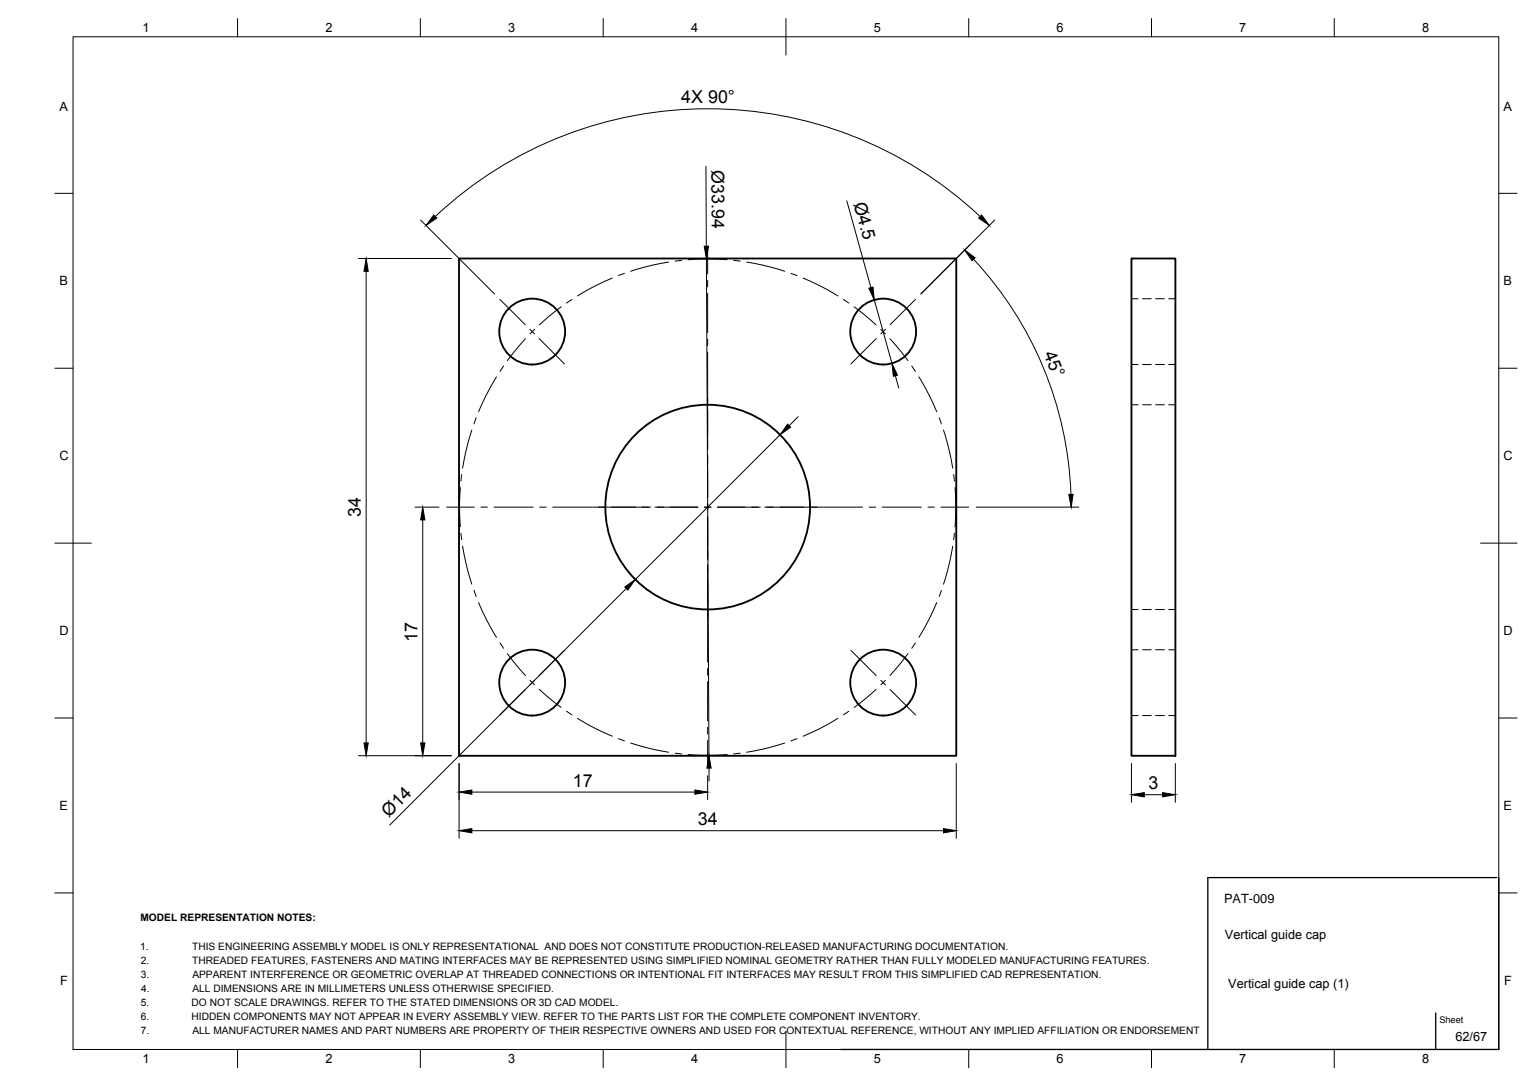
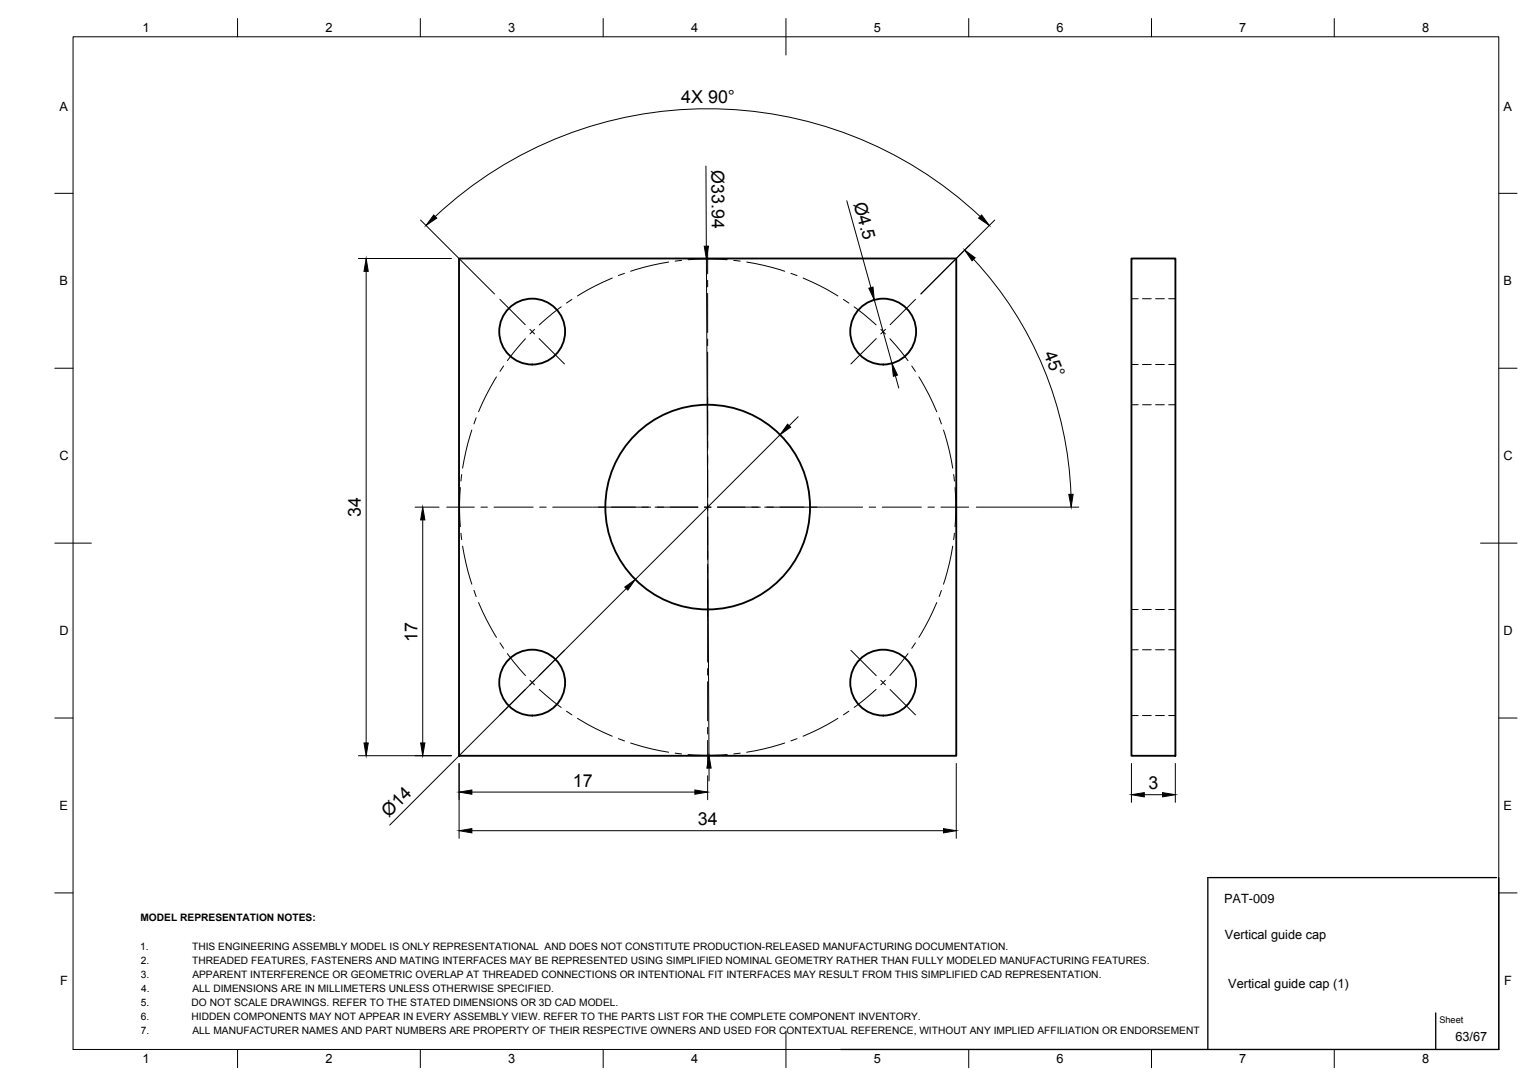
ISO-10303-21;
HEADER;
/* Generated by software containing ST-Developer
 * from STEP Tools, Inc. (www.steptools.com) 
 */

FILE_DESCRIPTION(
/* description */ ('Bell-crank linkage with push rods'),
/* implementation_level */ '2;1');

FILE_NAME(
/* name */ 'Vertical guide cap (1).step',
/* time_stamp */ '2026-10-28T03:25:15-07:00',
/* author */ (''),
/* organization */ (''),
/* preprocessor_version */ 'ST-DEVELOPER v20.2',
/* originating_system */ 'Autodesk Translation Framework v15.17.0.0',
/* authorisation */ '');

FILE_SCHEMA (('AUTOMOTIVE_DESIGN { 1 0 10303 214 3 1 1 }'));
ENDSEC;

DATA;
#10=MECHANICAL_DESIGN_GEOMETRIC_PRESENTATION_REPRESENTATION('',(#658),#16678);
#542=SHAPE_REPRESENTATION_RELATIONSHIP('SRR','None',#16964,#596);
#596=ADVANCED_BREP_SHAPE_REPRESENTATION('',(#718),#16669);
#658=STYLED_ITEM('',(#17277),#718);
#718=MANIFOLD_SOLID_BREP('Body1',#8850);
#935=FACE_BOUND('',#2434,.T.);
#936=FACE_BOUND('',#2435,.T.);
#937=FACE_BOUND('',#2436,.T.);
#938=FACE_BOUND('',#2437,.T.);
#939=FACE_BOUND('',#2438,.T.);
#940=FACE_BOUND('',#2441,.T.);
#941=FACE_BOUND('',#2442,.T.);
#942=FACE_BOUND('',#2443,.T.);
#943=FACE_BOUND('',#2444,.T.);
#944=FACE_BOUND('',#2445,.T.);
#1202=PLANE('',#10415);
#1203=PLANE('',#10416);
#1204=PLANE('',#10417);
#1205=PLANE('',#10418);
#1206=PLANE('',#10419);
#1207=PLANE('',#10420);
#1696=FACE_OUTER_BOUND('',#2428,.T.);
#1697=FACE_OUTER_BOUND('',#2429,.T.);
#1698=FACE_OUTER_BOUND('',#2430,.T.);
#1699=FACE_OUTER_BOUND('',#2431,.T.);
#1700=FACE_OUTER_BOUND('',#2432,.T.);
#1701=FACE_OUTER_BOUND('',#2433,.T.);
#1702=FACE_OUTER_BOUND('',#2439,.T.);
#1703=FACE_OUTER_BOUND('',#2440,.T.);
#1704=FACE_OUTER_BOUND('',#2446,.T.);
#1705=FACE_OUTER_BOUND('',#2447,.T.);
#1706=FACE_OUTER_BOUND('',#2448,.T.);
#2428=EDGE_LOOP('',(#7797,#7798,#7799,#7800));
#2429=EDGE_LOOP('',(#7801,#7802,#7803,#7804));
#2430=EDGE_LOOP('',(#7805,#7806,#7807,#7808));
#2431=EDGE_LOOP('',(#7809,#7810,#7811,#7812));
#2432=EDGE_LOOP('',(#7813,#7814,#7815,#7816));
#2433=EDGE_LOOP('',(#7817,#7818,#7819,#7820));
#2434=EDGE_LOOP('',(#7821));
#2435=EDGE_LOOP('',(#7822));
#2436=EDGE_LOOP('',(#7823));
#2437=EDGE_LOOP('',(#7824));
#2438=EDGE_LOOP('',(#7825));
#2439=EDGE_LOOP('',(#7826,#7827,#7828,#7829));
#2440=EDGE_LOOP('',(#7830,#7831,#7832,#7833));
#2441=EDGE_LOOP('',(#7834));
#2442=EDGE_LOOP('',(#7835));
#2443=EDGE_LOOP('',(#7836));
#2444=EDGE_LOOP('',(#7837));
#2445=EDGE_LOOP('',(#7838));
#2446=EDGE_LOOP('',(#7839,#7840,#7841,#7842));
#2447=EDGE_LOOP('',(#7843,#7844,#7845,#7846));
#2448=EDGE_LOOP('',(#7847,#7848,#7849,#7850));
#3005=LINE('',#16160,#3554);
#3006=LINE('',#16166,#3555);
#3007=LINE('',#16172,#3556);
#3008=LINE('',#16178,#3557);
#3009=LINE('',#16184,#3558);
#3010=LINE('',#16189,#3559);
#3011=LINE('',#16191,#3560);
#3012=LINE('',#16193,#3561);
#3013=LINE('',#16194,#3562);
#3014=LINE('',#16197,#3563);
#3015=LINE('',#16199,#3564);
#3016=LINE('',#16200,#3565);
#3017=LINE('',#16203,#3566);
#3018=LINE('',#16205,#3567);
#3019=LINE('',#16206,#3568);
#3020=LINE('',#16208,#3569);
#3021=LINE('',#16209,#3570);
#3554=VECTOR('',#12999,0.225);
#3555=VECTOR('',#13006,0.225);
#3556=VECTOR('',#13013,0.225);
#3557=VECTOR('',#13020,0.225);
#3558=VECTOR('',#13027,0.7);
#3559=VECTOR('',#13032,1.);
#3560=VECTOR('',#13033,1.);
#3561=VECTOR('',#13034,1.);
#3562=VECTOR('',#13035,1.);
#3563=VECTOR('',#13038,1.);
#3564=VECTOR('',#13039,1.);
#3565=VECTOR('',#13040,1.);
#3566=VECTOR('',#13043,1.);
#3567=VECTOR('',#13044,1.);
#3568=VECTOR('',#13045,1.);
#3569=VECTOR('',#13048,1.);
#3570=VECTOR('',#13049,1.);
#4061=CIRCLE('',#10401,0.225);
#4062=CIRCLE('',#10402,0.225);
#4063=CIRCLE('',#10404,0.225);
#4064=CIRCLE('',#10405,0.225);
#4065=CIRCLE('',#10407,0.225);
#4066=CIRCLE('',#10408,0.225);
#4067=CIRCLE('',#10410,0.225);
#4068=CIRCLE('',#10411,0.225);
#4069=CIRCLE('',#10413,0.7);
#4070=CIRCLE('',#10414,0.7);
#4744=VERTEX_POINT('',#16157);
#4745=VERTEX_POINT('',#16159);
#4746=VERTEX_POINT('',#16163);
#4747=VERTEX_POINT('',#16165);
#4748=VERTEX_POINT('',#16169);
#4749=VERTEX_POINT('',#16171);
#4750=VERTEX_POINT('',#16175);
#4751=VERTEX_POINT('',#16177);
#4752=VERTEX_POINT('',#16181);
#4753=VERTEX_POINT('',#16183);
#4754=VERTEX_POINT('',#16187);
#4755=VERTEX_POINT('',#16188);
#4756=VERTEX_POINT('',#16190);
#4757=VERTEX_POINT('',#16192);
#4758=VERTEX_POINT('',#16196);
#4759=VERTEX_POINT('',#16198);
#4760=VERTEX_POINT('',#16202);
#4761=VERTEX_POINT('',#16204);
#5776=EDGE_CURVE('',#4744,#4744,#4061,.T.);
#5777=EDGE_CURVE('',#4744,#4745,#3005,.T.);
#5778=EDGE_CURVE('',#4745,#4745,#4062,.T.);
#5779=EDGE_CURVE('',#4746,#4746,#4063,.T.);
#5780=EDGE_CURVE('',#4746,#4747,#3006,.T.);
#5781=EDGE_CURVE('',#4747,#4747,#4064,.T.);
#5782=EDGE_CURVE('',#4748,#4748,#4065,.T.);
#5783=EDGE_CURVE('',#4748,#4749,#3007,.T.);
#5784=EDGE_CURVE('',#4749,#4749,#4066,.T.);
#5785=EDGE_CURVE('',#4750,#4750,#4067,.T.);
#5786=EDGE_CURVE('',#4750,#4751,#3008,.T.);
#5787=EDGE_CURVE('',#4751,#4751,#4068,.T.);
#5788=EDGE_CURVE('',#4752,#4752,#4069,.T.);
#5789=EDGE_CURVE('',#4752,#4753,#3009,.T.);
#5790=EDGE_CURVE('',#4753,#4753,#4070,.T.);
#5791=EDGE_CURVE('',#4754,#4755,#3010,.T.);
#5792=EDGE_CURVE('',#4755,#4756,#3011,.T.);
#5793=EDGE_CURVE('',#4757,#4756,#3012,.T.);
#5794=EDGE_CURVE('',#4754,#4757,#3013,.T.);
#5795=EDGE_CURVE('',#4758,#4754,#3014,.T.);
#5796=EDGE_CURVE('',#4759,#4757,#3015,.T.);
#5797=EDGE_CURVE('',#4758,#4759,#3016,.T.);
#5798=EDGE_CURVE('',#4760,#4758,#3017,.T.);
#5799=EDGE_CURVE('',#4761,#4759,#3018,.T.);
#5800=EDGE_CURVE('',#4760,#4761,#3019,.T.);
#5801=EDGE_CURVE('',#4755,#4760,#3020,.T.);
#5802=EDGE_CURVE('',#4756,#4761,#3021,.T.);
#7797=ORIENTED_EDGE('',*,*,#5776,.F.);
#7798=ORIENTED_EDGE('',*,*,#5777,.T.);
#7799=ORIENTED_EDGE('',*,*,#5778,.F.);
#7800=ORIENTED_EDGE('',*,*,#5777,.F.);
#7801=ORIENTED_EDGE('',*,*,#5779,.F.);
#7802=ORIENTED_EDGE('',*,*,#5780,.T.);
#7803=ORIENTED_EDGE('',*,*,#5781,.F.);
#7804=ORIENTED_EDGE('',*,*,#5780,.F.);
#7805=ORIENTED_EDGE('',*,*,#5782,.F.);
#7806=ORIENTED_EDGE('',*,*,#5783,.T.);
#7807=ORIENTED_EDGE('',*,*,#5784,.F.);
#7808=ORIENTED_EDGE('',*,*,#5783,.F.);
#7809=ORIENTED_EDGE('',*,*,#5785,.F.);
#7810=ORIENTED_EDGE('',*,*,#5786,.T.);
#7811=ORIENTED_EDGE('',*,*,#5787,.F.);
#7812=ORIENTED_EDGE('',*,*,#5786,.F.);
#7813=ORIENTED_EDGE('',*,*,#5788,.F.);
#7814=ORIENTED_EDGE('',*,*,#5789,.T.);
#7815=ORIENTED_EDGE('',*,*,#5790,.F.);
#7816=ORIENTED_EDGE('',*,*,#5789,.F.);
#7817=ORIENTED_EDGE('',*,*,#5791,.T.);
#7818=ORIENTED_EDGE('',*,*,#5792,.T.);
#7819=ORIENTED_EDGE('',*,*,#5793,.F.);
#7820=ORIENTED_EDGE('',*,*,#5794,.F.);
#7821=ORIENTED_EDGE('',*,*,#5790,.T.);
#7822=ORIENTED_EDGE('',*,*,#5787,.T.);
#7823=ORIENTED_EDGE('',*,*,#5784,.T.);
#7824=ORIENTED_EDGE('',*,*,#5781,.T.);
#7825=ORIENTED_EDGE('',*,*,#5778,.T.);
#7826=ORIENTED_EDGE('',*,*,#5795,.T.);
#7827=ORIENTED_EDGE('',*,*,#5794,.T.);
#7828=ORIENTED_EDGE('',*,*,#5796,.F.);
#7829=ORIENTED_EDGE('',*,*,#5797,.F.);
#7830=ORIENTED_EDGE('',*,*,#5798,.T.);
#7831=ORIENTED_EDGE('',*,*,#5797,.T.);
#7832=ORIENTED_EDGE('',*,*,#5799,.F.);
#7833=ORIENTED_EDGE('',*,*,#5800,.F.);
#7834=ORIENTED_EDGE('',*,*,#5788,.T.);
#7835=ORIENTED_EDGE('',*,*,#5785,.T.);
#7836=ORIENTED_EDGE('',*,*,#5782,.T.);
#7837=ORIENTED_EDGE('',*,*,#5779,.T.);
#7838=ORIENTED_EDGE('',*,*,#5776,.T.);
#7839=ORIENTED_EDGE('',*,*,#5801,.T.);
#7840=ORIENTED_EDGE('',*,*,#5800,.T.);
#7841=ORIENTED_EDGE('',*,*,#5802,.F.);
#7842=ORIENTED_EDGE('',*,*,#5792,.F.);
#7843=ORIENTED_EDGE('',*,*,#5802,.T.);
#7844=ORIENTED_EDGE('',*,*,#5799,.T.);
#7845=ORIENTED_EDGE('',*,*,#5796,.T.);
#7846=ORIENTED_EDGE('',*,*,#5793,.T.);
#7847=ORIENTED_EDGE('',*,*,#5801,.F.);
#7848=ORIENTED_EDGE('',*,*,#5791,.F.);
#7849=ORIENTED_EDGE('',*,*,#5795,.F.);
#7850=ORIENTED_EDGE('',*,*,#5798,.F.);
#8247=CYLINDRICAL_SURFACE('',#10400,0.225);
#8248=CYLINDRICAL_SURFACE('',#10403,0.225);
#8249=CYLINDRICAL_SURFACE('',#10406,0.225);
#8250=CYLINDRICAL_SURFACE('',#10409,0.225);
#8251=CYLINDRICAL_SURFACE('',#10412,0.7);
#8721=ADVANCED_FACE('',(#1696),#8247,.F.);
#8722=ADVANCED_FACE('',(#1697),#8248,.F.);
#8723=ADVANCED_FACE('',(#1698),#8249,.F.);
#8724=ADVANCED_FACE('',(#1699),#8250,.F.);
#8725=ADVANCED_FACE('',(#1700),#8251,.F.);
#8726=ADVANCED_FACE('',(#1701,#935,#936,#937,#938,#939),#1202,.T.);
#8727=ADVANCED_FACE('',(#1702),#1203,.T.);
#8728=ADVANCED_FACE('',(#1703,#940,#941,#942,#943,#944),#1204,.T.);
#8729=ADVANCED_FACE('',(#1704),#1205,.T.);
#8730=ADVANCED_FACE('',(#1705),#1206,.T.);
#8731=ADVANCED_FACE('',(#1706),#1207,.F.);
#8850=CLOSED_SHELL('',(#8721,#8722,#8723,#8724,#8725,#8726,#8727,#8728,
#8729,#8730,#8731));
#10399=AXIS2_PLACEMENT_3D('',#16155,#12993,#12994);
#10400=AXIS2_PLACEMENT_3D('',#16156,#12995,#12996);
#10401=AXIS2_PLACEMENT_3D('',#16158,#12997,#12998);
#10402=AXIS2_PLACEMENT_3D('',#16161,#13000,#13001);
#10403=AXIS2_PLACEMENT_3D('',#16162,#13002,#13003);
#10404=AXIS2_PLACEMENT_3D('',#16164,#13004,#13005);
#10405=AXIS2_PLACEMENT_3D('',#16167,#13007,#13008);
#10406=AXIS2_PLACEMENT_3D('',#16168,#13009,#13010);
#10407=AXIS2_PLACEMENT_3D('',#16170,#13011,#13012);
#10408=AXIS2_PLACEMENT_3D('',#16173,#13014,#13015);
#10409=AXIS2_PLACEMENT_3D('',#16174,#13016,#13017);
#10410=AXIS2_PLACEMENT_3D('',#16176,#13018,#13019);
#10411=AXIS2_PLACEMENT_3D('',#16179,#13021,#13022);
#10412=AXIS2_PLACEMENT_3D('',#16180,#13023,#13024);
#10413=AXIS2_PLACEMENT_3D('',#16182,#13025,#13026);
#10414=AXIS2_PLACEMENT_3D('',#16185,#13028,#13029);
#10415=AXIS2_PLACEMENT_3D('',#16186,#13030,#13031);
#10416=AXIS2_PLACEMENT_3D('',#16195,#13036,#13037);
#10417=AXIS2_PLACEMENT_3D('',#16201,#13041,#13042);
#10418=AXIS2_PLACEMENT_3D('',#16207,#13046,#13047);
#10419=AXIS2_PLACEMENT_3D('',#16210,#13050,#13051);
#10420=AXIS2_PLACEMENT_3D('',#16211,#13052,#13053);
#12993=DIRECTION('axis',(0.,0.,1.));
#12994=DIRECTION('refdir',(1.,0.,0.));
#12995=DIRECTION('center_axis',(0.,1.,0.));
#12996=DIRECTION('ref_axis',(1.,0.,0.));
#12997=DIRECTION('center_axis',(0.,1.,0.));
#12998=DIRECTION('ref_axis',(1.,0.,0.));
#12999=DIRECTION('',(0.,1.,0.));
#13000=DIRECTION('center_axis',(0.,-1.,0.));
#13001=DIRECTION('ref_axis',(1.,0.,0.));
#13002=DIRECTION('center_axis',(0.,1.,0.));
#13003=DIRECTION('ref_axis',(1.,0.,0.));
#13004=DIRECTION('center_axis',(0.,1.,0.));
#13005=DIRECTION('ref_axis',(1.,0.,0.));
#13006=DIRECTION('',(0.,1.,0.));
#13007=DIRECTION('center_axis',(0.,-1.,0.));
#13008=DIRECTION('ref_axis',(1.,0.,0.));
#13009=DIRECTION('center_axis',(0.,1.,0.));
#13010=DIRECTION('ref_axis',(1.,0.,0.));
#13011=DIRECTION('center_axis',(0.,1.,0.));
#13012=DIRECTION('ref_axis',(1.,0.,0.));
#13013=DIRECTION('',(0.,1.,0.));
#13014=DIRECTION('center_axis',(0.,-1.,0.));
#13015=DIRECTION('ref_axis',(1.,0.,0.));
#13016=DIRECTION('center_axis',(0.,1.,0.));
#13017=DIRECTION('ref_axis',(1.,0.,0.));
#13018=DIRECTION('center_axis',(0.,1.,0.));
#13019=DIRECTION('ref_axis',(1.,0.,0.));
#13020=DIRECTION('',(0.,1.,0.));
#13021=DIRECTION('center_axis',(0.,-1.,0.));
#13022=DIRECTION('ref_axis',(1.,0.,0.));
#13023=DIRECTION('center_axis',(0.,1.,0.));
#13024=DIRECTION('ref_axis',(1.,0.,0.));
#13025=DIRECTION('center_axis',(0.,1.,0.));
#13026=DIRECTION('ref_axis',(1.,0.,0.));
#13027=DIRECTION('',(0.,1.,0.));
#13028=DIRECTION('center_axis',(0.,-1.,0.));
#13029=DIRECTION('ref_axis',(1.,0.,0.));
#13030=DIRECTION('center_axis',(0.,1.,0.));
#13031=DIRECTION('ref_axis',(-1.,0.,0.));
#13032=DIRECTION('',(-1.,0.,0.));
#13033=DIRECTION('',(0.,0.,1.));
#13034=DIRECTION('',(-1.,0.,0.));
#13035=DIRECTION('',(0.,0.,1.));
#13036=DIRECTION('center_axis',(1.,0.,0.));
#13037=DIRECTION('ref_axis',(0.,1.,0.));
#13038=DIRECTION('',(0.,1.,0.));
#13039=DIRECTION('',(0.,1.,0.));
#13040=DIRECTION('',(0.,0.,1.));
#13041=DIRECTION('center_axis',(0.,-1.,0.));
#13042=DIRECTION('ref_axis',(1.,0.,0.));
#13043=DIRECTION('',(1.,0.,0.));
#13044=DIRECTION('',(1.,0.,0.));
#13045=DIRECTION('',(0.,0.,1.));
#13046=DIRECTION('center_axis',(-1.,0.,0.));
#13047=DIRECTION('ref_axis',(0.,-1.,0.));
#13048=DIRECTION('',(0.,-1.,0.));
#13049=DIRECTION('',(0.,-1.,0.));
#13050=DIRECTION('center_axis',(0.,0.,1.));
#13051=DIRECTION('ref_axis',(1.,0.,0.));
#13052=DIRECTION('center_axis',(0.,0.,1.));
#13053=DIRECTION('ref_axis',(1.,0.,0.));
#16155=CARTESIAN_POINT('',(0.,0.,0.));
#16156=CARTESIAN_POINT('Origin',(5.2,13.4,2.8));
#16157=CARTESIAN_POINT('',(4.975,13.5,2.8));
#16158=CARTESIAN_POINT('Origin',(5.2,13.5,2.8));
#16159=CARTESIAN_POINT('',(4.975,13.8,2.8));
#16160=CARTESIAN_POINT('',(4.975,13.4,2.8));
#16161=CARTESIAN_POINT('Origin',(5.2,13.8,2.8));
#16162=CARTESIAN_POINT('Origin',(2.8,13.4,5.2));
#16163=CARTESIAN_POINT('',(2.575,13.5,5.2));
#16164=CARTESIAN_POINT('Origin',(2.8,13.5,5.2));
#16165=CARTESIAN_POINT('',(2.575,13.8,5.2));
#16166=CARTESIAN_POINT('',(2.575,13.4,5.2));
#16167=CARTESIAN_POINT('Origin',(2.8,13.8,5.2));
#16168=CARTESIAN_POINT('Origin',(2.8,13.4,2.8));
#16169=CARTESIAN_POINT('',(2.575,13.5,2.8));
#16170=CARTESIAN_POINT('Origin',(2.8,13.5,2.8));
#16171=CARTESIAN_POINT('',(2.575,13.8,2.8));
#16172=CARTESIAN_POINT('',(2.575,13.4,2.8));
#16173=CARTESIAN_POINT('Origin',(2.8,13.8,2.8));
#16174=CARTESIAN_POINT('Origin',(5.2,13.4,5.2));
#16175=CARTESIAN_POINT('',(4.975,13.5,5.2));
#16176=CARTESIAN_POINT('Origin',(5.2,13.5,5.2));
#16177=CARTESIAN_POINT('',(4.975,13.8,5.2));
#16178=CARTESIAN_POINT('',(4.975,13.4,5.2));
#16179=CARTESIAN_POINT('Origin',(5.2,13.8,5.2));
#16180=CARTESIAN_POINT('Origin',(4.,13.4,4.));
#16181=CARTESIAN_POINT('',(3.3,13.5,4.));
#16182=CARTESIAN_POINT('Origin',(4.,13.5,4.));
#16183=CARTESIAN_POINT('',(3.3,13.8,4.));
#16184=CARTESIAN_POINT('',(3.3,13.4,4.));
#16185=CARTESIAN_POINT('Origin',(4.,13.8,4.));
#16186=CARTESIAN_POINT('Origin',(5.7,13.8,2.3));
#16187=CARTESIAN_POINT('',(5.7,13.8,2.3));
#16188=CARTESIAN_POINT('',(2.3,13.8,2.3));
#16189=CARTESIAN_POINT('',(5.7,13.8,2.3));
#16190=CARTESIAN_POINT('',(2.3,13.8,5.7));
#16191=CARTESIAN_POINT('',(2.3,13.8,2.3));
#16192=CARTESIAN_POINT('',(5.7,13.8,5.7));
#16193=CARTESIAN_POINT('',(5.7,13.8,5.7));
#16194=CARTESIAN_POINT('',(5.7,13.8,2.3));
#16195=CARTESIAN_POINT('Origin',(5.7,13.5,2.3));
#16196=CARTESIAN_POINT('',(5.7,13.5,2.3));
#16197=CARTESIAN_POINT('',(5.7,13.5,2.3));
#16198=CARTESIAN_POINT('',(5.7,13.5,5.7));
#16199=CARTESIAN_POINT('',(5.7,13.5,5.7));
#16200=CARTESIAN_POINT('',(5.7,13.5,2.3));
#16201=CARTESIAN_POINT('Origin',(2.3,13.5,2.3));
#16202=CARTESIAN_POINT('',(2.3,13.5,2.3));
#16203=CARTESIAN_POINT('',(2.3,13.5,2.3));
#16204=CARTESIAN_POINT('',(2.3,13.5,5.7));
#16205=CARTESIAN_POINT('',(2.3,13.5,5.7));
#16206=CARTESIAN_POINT('',(2.3,13.5,2.3));
#16207=CARTESIAN_POINT('Origin',(2.3,13.8,2.3));
#16208=CARTESIAN_POINT('',(2.3,13.8,2.3));
#16209=CARTESIAN_POINT('',(2.3,13.8,5.7));
#16210=CARTESIAN_POINT('Origin',(4.,13.65,5.7));
#16211=CARTESIAN_POINT('Origin',(4.,13.65,2.3));
#16605=UNCERTAINTY_MEASURE_WITH_UNIT(LENGTH_MEASURE(0.001),#16679,
'DISTANCE_ACCURACY_VALUE',
'Maximum model space distance between geometric entities at asserted c
onnectivities');
#16614=UNCERTAINTY_MEASURE_WITH_UNIT(LENGTH_MEASURE(0.001),#16679,
'DISTANCE_ACCURACY_VALUE',
'Maximum model space distance between geometric entities at asserted c
onnectivities');
#16669=(
GEOMETRIC_REPRESENTATION_CONTEXT(3)
GLOBAL_UNCERTAINTY_ASSIGNED_CONTEXT((#16605))
GLOBAL_UNIT_ASSIGNED_CONTEXT((#16679,#16681,#16682))
REPRESENTATION_CONTEXT('','3D')
);
#16678=(
GEOMETRIC_REPRESENTATION_CONTEXT(3)
GLOBAL_UNCERTAINTY_ASSIGNED_CONTEXT((#16614))
GLOBAL_UNIT_ASSIGNED_CONTEXT((#16679,#16681,#16682))
REPRESENTATION_CONTEXT('','3D')
);
#16679=(
LENGTH_UNIT()
NAMED_UNIT(*)
SI_UNIT(.CENTI.,.METRE.)
);
#16681=(
NAMED_UNIT(*)
PLANE_ANGLE_UNIT()
SI_UNIT($,.RADIAN.)
);
#16682=(
NAMED_UNIT(*)
SI_UNIT($,.STERADIAN.)
SOLID_ANGLE_UNIT()
);
#16737=SHAPE_DEFINITION_REPRESENTATION(#16811,#16964);
#16811=PRODUCT_DEFINITION_SHAPE('',$,#17028);
#16964=SHAPE_REPRESENTATION('',(#10399),#16669);
#16973=PRODUCT_DEFINITION_CONTEXT('part definition',#17164,'design');
#17028=PRODUCT_DEFINITION('Vertical guide cap (1)',
'Vertical guide cap (1)',#17091,#16973);
#17091=PRODUCT_DEFINITION_FORMATION('',$,#17220);
#17164=APPLICATION_CONTEXT(
'Core Data for Automotive Mechanical Design Process');
#17165=PRODUCT_CONTEXT('part definition',#17164,'mechanical');
#17220=PRODUCT('Vertical guide cap (1)','Vertical guide cap (1)',
'Vertical guide cap (1)',(#17165));
#17271=COLOUR_RGB('Light Blue',0.38,0.62,0.78);
#17272=FILL_AREA_STYLE_COLOUR('',#17271);
#17273=FILL_AREA_STYLE('',(#17272));
#17274=SURFACE_STYLE_FILL_AREA(#17273);
#17275=SURFACE_SIDE_STYLE('',(#17274));
#17276=SURFACE_STYLE_USAGE(.BOTH.,#17275);
#17277=PRESENTATION_STYLE_ASSIGNMENT((#17276));
ENDSEC;
END-ISO-10303-21;
